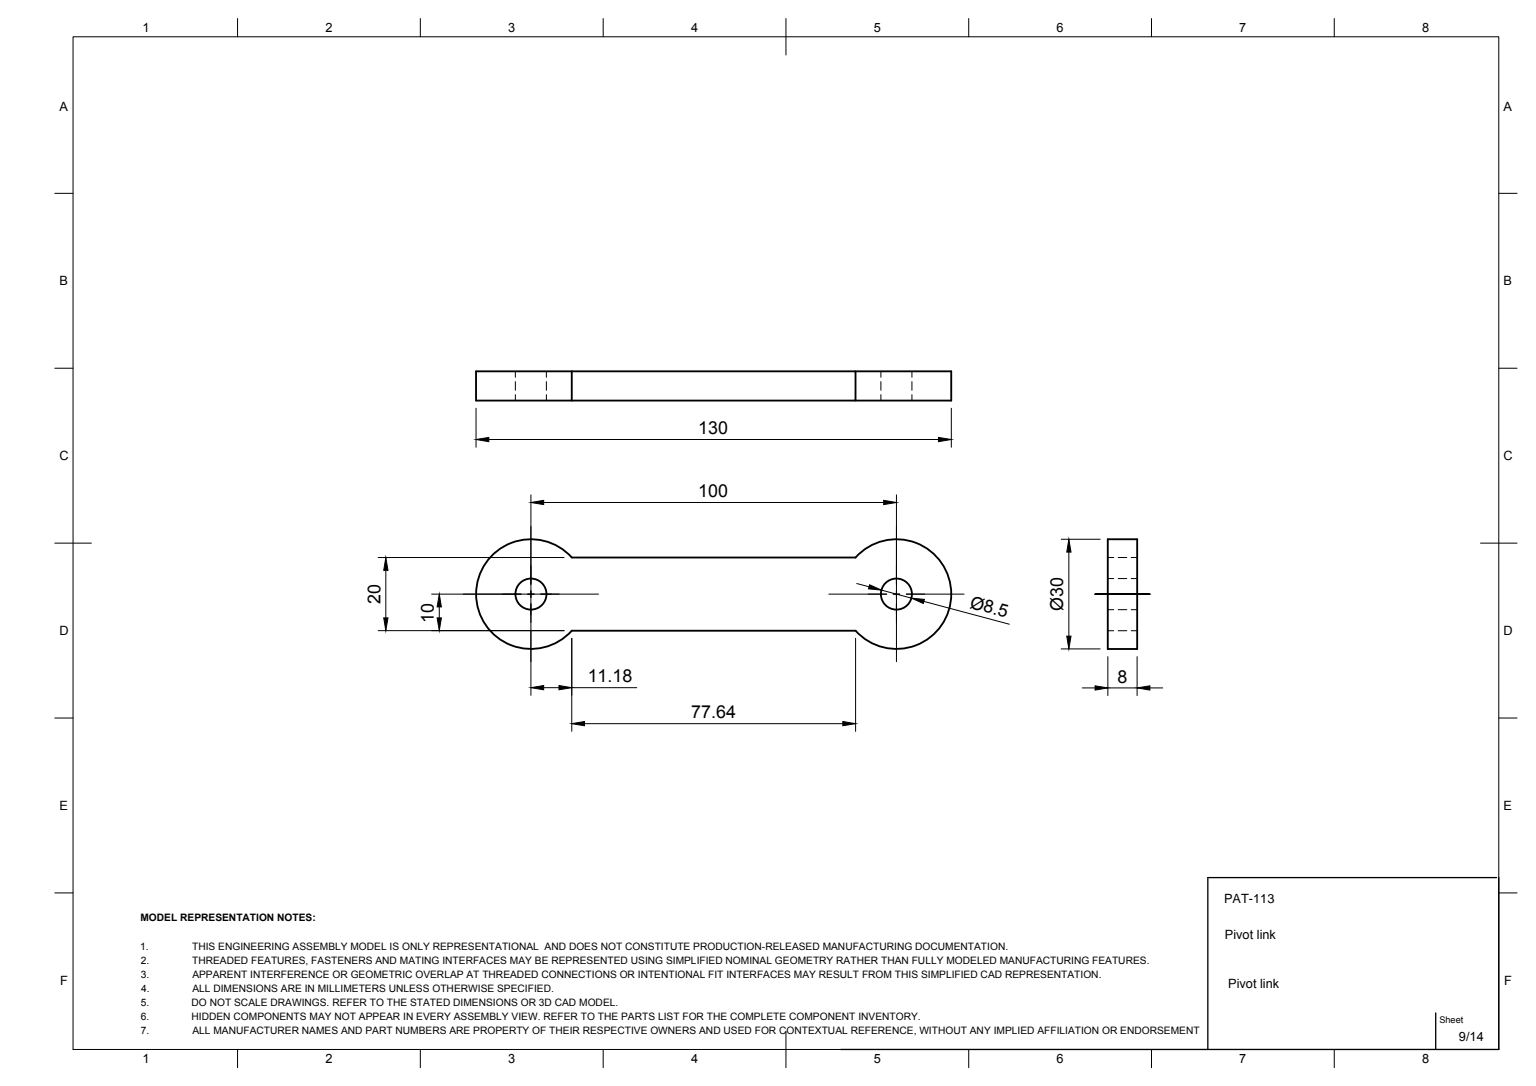
ISO-10303-21;
HEADER;
/* Generated by software containing ST-Developer
 * from STEP Tools, Inc. (www.steptools.com) 
 */

FILE_DESCRIPTION(
/* description */ ('Two-link friction support arm'),
/* implementation_level */ '2;1');

FILE_NAME(
/* name */ 'Pivot link.step',
/* time_stamp */ '2026-10-27T20:01:49-07:00',
/* author */ (''),
/* organization */ (''),
/* preprocessor_version */ 'ST-DEVELOPER v20.2',
/* originating_system */ 'Autodesk Translation Framework v15.17.0.0',
/* authorisation */ '');

FILE_SCHEMA (('AUTOMOTIVE_DESIGN { 1 0 10303 214 3 1 1 }'));
ENDSEC;

DATA;
#10=MECHANICAL_DESIGN_GEOMETRIC_PRESENTATION_REPRESENTATION('',(#200),#5492);
#178=SHAPE_REPRESENTATION_RELATIONSHIP('SRR','None',#5571,#189);
#189=ADVANCED_BREP_SHAPE_REPRESENTATION('',(#210),#5485);
#200=STYLED_ITEM('',(#5687),#210);
#210=MANIFOLD_SOLID_BREP('Body1',#3177);
#228=FACE_BOUND('',#652,.T.);
#229=FACE_BOUND('',#653,.T.);
#230=FACE_BOUND('',#657,.T.);
#231=FACE_BOUND('',#658,.T.);
#332=PLANE('',#3445);
#333=PLANE('',#3446);
#334=PLANE('',#3448);
#335=PLANE('',#3451);
#468=FACE_OUTER_BOUND('',#647,.T.);
#469=FACE_OUTER_BOUND('',#648,.T.);
#470=FACE_OUTER_BOUND('',#649,.T.);
#471=FACE_OUTER_BOUND('',#650,.T.);
#472=FACE_OUTER_BOUND('',#651,.T.);
#473=FACE_OUTER_BOUND('',#654,.T.);
#474=FACE_OUTER_BOUND('',#655,.T.);
#475=FACE_OUTER_BOUND('',#656,.T.);
#647=EDGE_LOOP('',(#2628,#2629,#2630,#2631));
#648=EDGE_LOOP('',(#2632,#2633,#2634,#2635));
#649=EDGE_LOOP('',(#2636,#2637,#2638,#2639));
#650=EDGE_LOOP('',(#2640,#2641,#2642,#2643));
#651=EDGE_LOOP('',(#2644,#2645,#2646,#2647));
#652=EDGE_LOOP('',(#2648));
#653=EDGE_LOOP('',(#2649));
#654=EDGE_LOOP('',(#2650,#2651,#2652,#2653));
#655=EDGE_LOOP('',(#2654,#2655,#2656,#2657));
#656=EDGE_LOOP('',(#2658,#2659,#2660,#2661));
#657=EDGE_LOOP('',(#2662));
#658=EDGE_LOOP('',(#2663));
#960=LINE('',#5034,#1273);
#961=LINE('',#5040,#1274);
#962=LINE('',#5045,#1275);
#963=LINE('',#5049,#1276);
#964=LINE('',#5053,#1277);
#965=LINE('',#5055,#1278);
#966=LINE('',#5056,#1279);
#967=LINE('',#5059,#1280);
#968=LINE('',#5063,#1281);
#969=LINE('',#5064,#1282);
#1273=VECTOR('',#4090,0.425);
#1274=VECTOR('',#4097,0.425000000000001);
#1275=VECTOR('',#4102,1.);
#1276=VECTOR('',#4105,1.);
#1277=VECTOR('',#4110,1.);
#1278=VECTOR('',#4111,1.);
#1279=VECTOR('',#4112,1.);
#1280=VECTOR('',#4115,1.);
#1281=VECTOR('',#4120,1.);
#1282=VECTOR('',#4121,1.);
#1391=CIRCLE('',#3437,0.425);
#1392=CIRCLE('',#3438,0.425);
#1393=CIRCLE('',#3440,0.425000000000001);
#1394=CIRCLE('',#3441,0.425000000000001);
#1395=CIRCLE('',#3443,1.5);
#1396=CIRCLE('',#3444,1.5);
#1397=CIRCLE('',#3447,1.5);
#1398=CIRCLE('',#3450,1.5);
#1611=VERTEX_POINT('',#5031);
#1612=VERTEX_POINT('',#5033);
#1613=VERTEX_POINT('',#5037);
#1614=VERTEX_POINT('',#5039);
#1615=VERTEX_POINT('',#5043);
#1616=VERTEX_POINT('',#5044);
#1617=VERTEX_POINT('',#5046);
#1618=VERTEX_POINT('',#5048);
#1619=VERTEX_POINT('',#5052);
#1620=VERTEX_POINT('',#5054);
#1621=VERTEX_POINT('',#5058);
#1622=VERTEX_POINT('',#5062);
#1968=EDGE_CURVE('',#1611,#1611,#1391,.T.);
#1969=EDGE_CURVE('',#1611,#1612,#960,.T.);
#1970=EDGE_CURVE('',#1612,#1612,#1392,.T.);
#1971=EDGE_CURVE('',#1613,#1613,#1393,.T.);
#1972=EDGE_CURVE('',#1613,#1614,#961,.T.);
#1973=EDGE_CURVE('',#1614,#1614,#1394,.T.);
#1974=EDGE_CURVE('',#1615,#1616,#962,.T.);
#1975=EDGE_CURVE('',#1617,#1615,#1395,.T.);
#1976=EDGE_CURVE('',#1618,#1617,#963,.T.);
#1977=EDGE_CURVE('',#1618,#1616,#1396,.T.);
#1978=EDGE_CURVE('',#1619,#1616,#964,.T.);
#1979=EDGE_CURVE('',#1620,#1619,#965,.T.);
#1980=EDGE_CURVE('',#1615,#1620,#966,.T.);
#1981=EDGE_CURVE('',#1618,#1621,#967,.T.);
#1982=EDGE_CURVE('',#1619,#1621,#1397,.T.);
#1983=EDGE_CURVE('',#1622,#1617,#968,.T.);
#1984=EDGE_CURVE('',#1621,#1622,#969,.T.);
#1985=EDGE_CURVE('',#1620,#1622,#1398,.T.);
#2628=ORIENTED_EDGE('',*,*,#1968,.F.);
#2629=ORIENTED_EDGE('',*,*,#1969,.T.);
#2630=ORIENTED_EDGE('',*,*,#1970,.F.);
#2631=ORIENTED_EDGE('',*,*,#1969,.F.);
#2632=ORIENTED_EDGE('',*,*,#1971,.F.);
#2633=ORIENTED_EDGE('',*,*,#1972,.T.);
#2634=ORIENTED_EDGE('',*,*,#1973,.F.);
#2635=ORIENTED_EDGE('',*,*,#1972,.F.);
#2636=ORIENTED_EDGE('',*,*,#1974,.F.);
#2637=ORIENTED_EDGE('',*,*,#1975,.F.);
#2638=ORIENTED_EDGE('',*,*,#1976,.F.);
#2639=ORIENTED_EDGE('',*,*,#1977,.T.);
#2640=ORIENTED_EDGE('',*,*,#1974,.T.);
#2641=ORIENTED_EDGE('',*,*,#1978,.F.);
#2642=ORIENTED_EDGE('',*,*,#1979,.F.);
#2643=ORIENTED_EDGE('',*,*,#1980,.F.);
#2644=ORIENTED_EDGE('',*,*,#1977,.F.);
#2645=ORIENTED_EDGE('',*,*,#1981,.T.);
#2646=ORIENTED_EDGE('',*,*,#1982,.F.);
#2647=ORIENTED_EDGE('',*,*,#1978,.T.);
#2648=ORIENTED_EDGE('',*,*,#1968,.T.);
#2649=ORIENTED_EDGE('',*,*,#1971,.T.);
#2650=ORIENTED_EDGE('',*,*,#1976,.T.);
#2651=ORIENTED_EDGE('',*,*,#1983,.F.);
#2652=ORIENTED_EDGE('',*,*,#1984,.F.);
#2653=ORIENTED_EDGE('',*,*,#1981,.F.);
#2654=ORIENTED_EDGE('',*,*,#1979,.T.);
#2655=ORIENTED_EDGE('',*,*,#1982,.T.);
#2656=ORIENTED_EDGE('',*,*,#1984,.T.);
#2657=ORIENTED_EDGE('',*,*,#1985,.F.);
#2658=ORIENTED_EDGE('',*,*,#1980,.T.);
#2659=ORIENTED_EDGE('',*,*,#1985,.T.);
#2660=ORIENTED_EDGE('',*,*,#1983,.T.);
#2661=ORIENTED_EDGE('',*,*,#1975,.T.);
#2662=ORIENTED_EDGE('',*,*,#1970,.T.);
#2663=ORIENTED_EDGE('',*,*,#1973,.T.);
#2977=CYLINDRICAL_SURFACE('',#3436,0.425);
#2978=CYLINDRICAL_SURFACE('',#3439,0.425000000000001);
#2979=CYLINDRICAL_SURFACE('',#3442,1.5);
#2980=CYLINDRICAL_SURFACE('',#3449,1.5);
#3099=ADVANCED_FACE('',(#468),#2977,.F.);
#3100=ADVANCED_FACE('',(#469),#2978,.F.);
#3101=ADVANCED_FACE('',(#470),#2979,.T.);
#3102=ADVANCED_FACE('',(#471),#332,.T.);
#3103=ADVANCED_FACE('',(#472,#228,#229),#333,.F.);
#3104=ADVANCED_FACE('',(#473),#334,.T.);
#3105=ADVANCED_FACE('',(#474),#2980,.T.);
#3106=ADVANCED_FACE('',(#475,#230,#231),#335,.T.);
#3177=CLOSED_SHELL('',(#3099,#3100,#3101,#3102,#3103,#3104,#3105,#3106));
#3435=AXIS2_PLACEMENT_3D('',#5029,#4084,#4085);
#3436=AXIS2_PLACEMENT_3D('',#5030,#4086,#4087);
#3437=AXIS2_PLACEMENT_3D('',#5032,#4088,#4089);
#3438=AXIS2_PLACEMENT_3D('',#5035,#4091,#4092);
#3439=AXIS2_PLACEMENT_3D('',#5036,#4093,#4094);
#3440=AXIS2_PLACEMENT_3D('',#5038,#4095,#4096);
#3441=AXIS2_PLACEMENT_3D('',#5041,#4098,#4099);
#3442=AXIS2_PLACEMENT_3D('',#5042,#4100,#4101);
#3443=AXIS2_PLACEMENT_3D('',#5047,#4103,#4104);
#3444=AXIS2_PLACEMENT_3D('',#5050,#4106,#4107);
#3445=AXIS2_PLACEMENT_3D('',#5051,#4108,#4109);
#3446=AXIS2_PLACEMENT_3D('',#5057,#4113,#4114);
#3447=AXIS2_PLACEMENT_3D('',#5060,#4116,#4117);
#3448=AXIS2_PLACEMENT_3D('',#5061,#4118,#4119);
#3449=AXIS2_PLACEMENT_3D('',#5065,#4122,#4123);
#3450=AXIS2_PLACEMENT_3D('',#5066,#4124,#4125);
#3451=AXIS2_PLACEMENT_3D('',#5067,#4126,#4127);
#4084=DIRECTION('axis',(0.,0.,1.));
#4085=DIRECTION('refdir',(1.,0.,0.));
#4086=DIRECTION('center_axis',(0.,1.,0.));
#4087=DIRECTION('ref_axis',(1.,0.,0.));
#4088=DIRECTION('center_axis',(0.,1.,0.));
#4089=DIRECTION('ref_axis',(1.,0.,0.));
#4090=DIRECTION('',(0.,1.,0.));
#4091=DIRECTION('center_axis',(0.,-1.,0.));
#4092=DIRECTION('ref_axis',(1.,0.,0.));
#4093=DIRECTION('center_axis',(0.,1.,0.));
#4094=DIRECTION('ref_axis',(1.,0.,0.));
#4095=DIRECTION('center_axis',(0.,1.,0.));
#4096=DIRECTION('ref_axis',(1.,0.,0.));
#4097=DIRECTION('',(0.,1.,0.));
#4098=DIRECTION('center_axis',(0.,-1.,0.));
#4099=DIRECTION('ref_axis',(1.,0.,0.));
#4100=DIRECTION('center_axis',(0.,1.,0.));
#4101=DIRECTION('ref_axis',(1.,0.,0.));
#4102=DIRECTION('',(0.,-1.,0.));
#4103=DIRECTION('center_axis',(0.,1.,0.));
#4104=DIRECTION('ref_axis',(1.,0.,0.));
#4105=DIRECTION('',(0.,1.,0.));
#4106=DIRECTION('center_axis',(0.,1.,0.));
#4107=DIRECTION('ref_axis',(1.,0.,0.));
#4108=DIRECTION('center_axis',(0.,0.,-1.));
#4109=DIRECTION('ref_axis',(-1.,0.,0.));
#4110=DIRECTION('',(1.,0.,0.));
#4111=DIRECTION('',(0.,-1.,0.));
#4112=DIRECTION('',(-1.,0.,0.));
#4113=DIRECTION('center_axis',(0.,1.,0.));
#4114=DIRECTION('ref_axis',(1.,0.,0.));
#4115=DIRECTION('',(-1.,0.,0.));
#4116=DIRECTION('center_axis',(0.,1.,0.));
#4117=DIRECTION('ref_axis',(1.,0.,0.));
#4118=DIRECTION('center_axis',(0.,0.,1.));
#4119=DIRECTION('ref_axis',(1.,0.,0.));
#4120=DIRECTION('',(1.,0.,0.));
#4121=DIRECTION('',(0.,1.,0.));
#4122=DIRECTION('center_axis',(0.,1.,0.));
#4123=DIRECTION('ref_axis',(-1.,0.,-1.22464679914735E-16));
#4124=DIRECTION('center_axis',(0.,1.,0.));
#4125=DIRECTION('ref_axis',(1.,0.,0.));
#4126=DIRECTION('center_axis',(0.,1.,0.));
#4127=DIRECTION('ref_axis',(1.,0.,0.));
#5029=CARTESIAN_POINT('',(0.,0.,0.));
#5030=CARTESIAN_POINT('Origin',(5.,0.06,8.));
#5031=CARTESIAN_POINT('',(4.575,0.16,8.));
#5032=CARTESIAN_POINT('Origin',(5.,0.16,8.));
#5033=CARTESIAN_POINT('',(4.575,0.96,8.));
#5034=CARTESIAN_POINT('',(4.575,0.06,8.));
#5035=CARTESIAN_POINT('Origin',(5.,0.96,8.));
#5036=CARTESIAN_POINT('Origin',(15.,0.06,8.));
#5037=CARTESIAN_POINT('',(14.575,0.16,8.));
#5038=CARTESIAN_POINT('Origin',(15.,0.16,8.));
#5039=CARTESIAN_POINT('',(14.575,0.96,8.));
#5040=CARTESIAN_POINT('',(14.575,0.06,8.));
#5041=CARTESIAN_POINT('Origin',(15.,0.96,8.));
#5042=CARTESIAN_POINT('Origin',(15.,0.16,8.));
#5043=CARTESIAN_POINT('',(13.8819660112501,0.96,7.));
#5044=CARTESIAN_POINT('',(13.8819660112501,0.16,7.));
#5045=CARTESIAN_POINT('',(13.8819660112501,0.16,7.));
#5046=CARTESIAN_POINT('',(13.8819660112501,0.96,9.));
#5047=CARTESIAN_POINT('Origin',(15.,0.96,8.));
#5048=CARTESIAN_POINT('',(13.8819660112501,0.16,9.));
#5049=CARTESIAN_POINT('',(13.8819660112501,0.16,9.));
#5050=CARTESIAN_POINT('Origin',(15.,0.16,8.));
#5051=CARTESIAN_POINT('Origin',(15.,0.16,7.));
#5052=CARTESIAN_POINT('',(6.11803398874989,0.16,7.));
#5053=CARTESIAN_POINT('',(5.,0.16,7.));
#5054=CARTESIAN_POINT('',(6.11803398874989,0.96,7.));
#5055=CARTESIAN_POINT('',(6.11803398874989,0.16,7.));
#5056=CARTESIAN_POINT('',(5.,0.96,7.));
#5057=CARTESIAN_POINT('Origin',(5.,0.16,8.));
#5058=CARTESIAN_POINT('',(6.11803398874989,0.16,9.));
#5059=CARTESIAN_POINT('',(15.,0.16,9.));
#5060=CARTESIAN_POINT('Origin',(5.,0.16,8.));
#5061=CARTESIAN_POINT('Origin',(5.,0.16,9.));
#5062=CARTESIAN_POINT('',(6.11803398874989,0.96,9.));
#5063=CARTESIAN_POINT('',(15.,0.96,9.));
#5064=CARTESIAN_POINT('',(6.11803398874989,0.16,9.));
#5065=CARTESIAN_POINT('Origin',(5.,0.16,8.));
#5066=CARTESIAN_POINT('Origin',(5.,0.96,8.));
#5067=CARTESIAN_POINT('Origin',(5.,0.96,8.));
#5468=UNCERTAINTY_MEASURE_WITH_UNIT(LENGTH_MEASURE(0.001),#5493,
'DISTANCE_ACCURACY_VALUE',
'Maximum model space distance between geometric entities at asserted c
onnectivities');
#5475=UNCERTAINTY_MEASURE_WITH_UNIT(LENGTH_MEASURE(0.001),#5493,
'DISTANCE_ACCURACY_VALUE',
'Maximum model space distance between geometric entities at asserted c
onnectivities');
#5485=(
GEOMETRIC_REPRESENTATION_CONTEXT(3)
GLOBAL_UNCERTAINTY_ASSIGNED_CONTEXT((#5468))
GLOBAL_UNIT_ASSIGNED_CONTEXT((#5493,#5495,#5496))
REPRESENTATION_CONTEXT('','3D')
);
#5492=(
GEOMETRIC_REPRESENTATION_CONTEXT(3)
GLOBAL_UNCERTAINTY_ASSIGNED_CONTEXT((#5475))
GLOBAL_UNIT_ASSIGNED_CONTEXT((#5493,#5495,#5496))
REPRESENTATION_CONTEXT('','3D')
);
#5493=(
LENGTH_UNIT()
NAMED_UNIT(*)
SI_UNIT(.CENTI.,.METRE.)
);
#5495=(
NAMED_UNIT(*)
PLANE_ANGLE_UNIT()
SI_UNIT($,.RADIAN.)
);
#5496=(
NAMED_UNIT(*)
SI_UNIT($,.STERADIAN.)
SOLID_ANGLE_UNIT()
);
#5506=SHAPE_DEFINITION_REPRESENTATION(#5522,#5571);
#5522=PRODUCT_DEFINITION_SHAPE('',$,#5588);
#5571=SHAPE_REPRESENTATION('',(#3435),#5485);
#5578=PRODUCT_DEFINITION_CONTEXT('part definition',#5628,'design');
#5588=PRODUCT_DEFINITION('Pivot link','Pivot link',#5604,#5578);
#5604=PRODUCT_DEFINITION_FORMATION('',$,#5639);
#5628=APPLICATION_CONTEXT(
'Core Data for Automotive Mechanical Design Process');
#5629=PRODUCT_CONTEXT('part definition',#5628,'mechanical');
#5639=PRODUCT('Pivot link','Pivot link','Pivot link',(#5629));
#5681=COLOUR_RGB('Light Blue',0.38,0.62,0.78);
#5682=FILL_AREA_STYLE_COLOUR('',#5681);
#5683=FILL_AREA_STYLE('',(#5682));
#5684=SURFACE_STYLE_FILL_AREA(#5683);
#5685=SURFACE_SIDE_STYLE('',(#5684));
#5686=SURFACE_STYLE_USAGE(.BOTH.,#5685);
#5687=PRESENTATION_STYLE_ASSIGNMENT((#5686));
ENDSEC;
END-ISO-10303-21;
